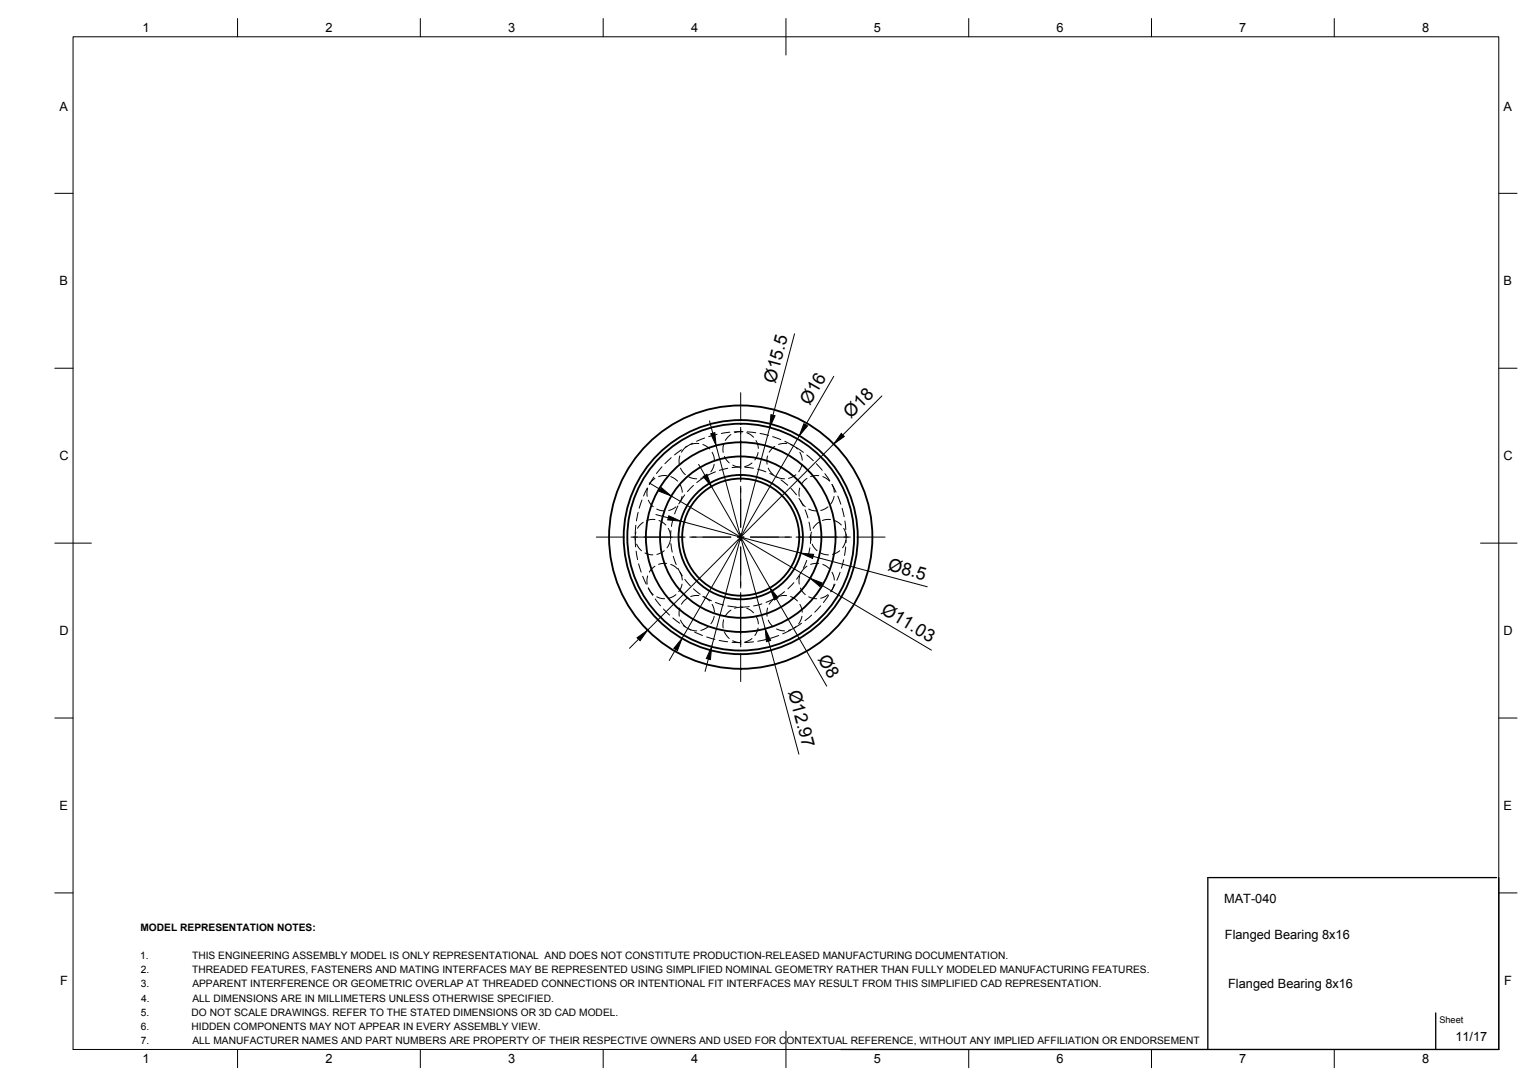
ISO-10303-21;
HEADER;
/* Generated by software containing ST-Developer
 * from STEP Tools, Inc. (www.steptools.com) 
 */

FILE_DESCRIPTION(
/* description */ ('STEP AP214'),
/* implementation_level */ '2;1');

FILE_NAME(
/* name */ 'Flanged Bearing 8x16.step',
/* time_stamp */ '2026-11-14T21:53:28-08:00',
/* author */ (''),
/* organization */ (''),
/* preprocessor_version */ 'ST-DEVELOPER v20.2',
/* originating_system */ 'Autodesk Translation Framework v15.17.0.0',
/* authorisation */ '');

FILE_SCHEMA (('AUTOMOTIVE_DESIGN { 1 0 10303 214 3 1 1 }'));
ENDSEC;

DATA;
#10=MECHANICAL_DESIGN_GEOMETRIC_PRESENTATION_REPRESENTATION('',(#333,#334,#335,#336,#337,#338,#339,#340,#341,#342,#343,#344,#345,#346,#347,#348),#20176);
#215=CONICAL_SURFACE('',#12015,4.25,0.785398163397453);
#216=CONICAL_SURFACE('',#12021,4.,0.785398163397443);
#217=CONICAL_SURFACE('',#12084,8.,0.785398163397446);
#229=TOROIDAL_SURFACE('',#12011,6.,1.21175743903915);
#230=TOROIDAL_SURFACE('',#12075,6.,1.21175743903915);
#252=SPHERICAL_SURFACE('',#12029,1.21175743903915);
#253=SPHERICAL_SURFACE('',#12031,1.21175743903915);
#254=SPHERICAL_SURFACE('',#12033,1.21175743903915);
#255=SPHERICAL_SURFACE('',#12035,1.21175743903915);
#256=SPHERICAL_SURFACE('',#12037,1.21175743903915);
#257=SPHERICAL_SURFACE('',#12039,1.21175743903915);
#258=SPHERICAL_SURFACE('',#12041,1.21175743903915);
#259=SPHERICAL_SURFACE('',#12043,1.21175743903915);
#260=SPHERICAL_SURFACE('',#12045,1.21175743903915);
#261=SPHERICAL_SURFACE('',#12047,1.21175743903915);
#262=SPHERICAL_SURFACE('',#12049,1.21175743903915);
#263=SPHERICAL_SURFACE('',#12051,1.21175743903915);
#301=SHAPE_REPRESENTATION_RELATIONSHIP('SRR','None',#20265,#313);
#313=ADVANCED_BREP_SHAPE_REPRESENTATION('',(#360,#361,#362,#363,#364,#365,
#366,#367,#368,#369,#370,#371,#372,#373,#374,#375),#20171);
#333=STYLED_ITEM('',(#20338),#360);
#334=STYLED_ITEM('',(#20338),#361);
#335=STYLED_ITEM('',(#20338),#362);
#336=STYLED_ITEM('',(#20338),#363);
#337=STYLED_ITEM('',(#20338),#364);
#338=STYLED_ITEM('',(#20338),#365);
#339=STYLED_ITEM('',(#20338),#366);
#340=STYLED_ITEM('',(#20338),#367);
#341=STYLED_ITEM('',(#20338),#368);
#342=STYLED_ITEM('',(#20338),#369);
#343=STYLED_ITEM('',(#20338),#370);
#344=STYLED_ITEM('',(#20338),#371);
#345=STYLED_ITEM('',(#20338),#372);
#346=STYLED_ITEM('',(#20338),#373);
#347=STYLED_ITEM('',(#20338),#374);
#348=STYLED_ITEM('',(#20338),#375);
#360=MANIFOLD_SOLID_BREP('Body1',#10951);
#361=MANIFOLD_SOLID_BREP('Body2',#10952);
#362=MANIFOLD_SOLID_BREP('Body3',#10953);
#363=MANIFOLD_SOLID_BREP('Body4',#10954);
#364=MANIFOLD_SOLID_BREP('Body5',#10955);
#365=MANIFOLD_SOLID_BREP('Body6',#10956);
#366=MANIFOLD_SOLID_BREP('Body7',#10957);
#367=MANIFOLD_SOLID_BREP('Body8',#10958);
#368=MANIFOLD_SOLID_BREP('Body9',#10959);
#369=MANIFOLD_SOLID_BREP('Body10',#10960);
#370=MANIFOLD_SOLID_BREP('Body11',#10961);
#371=MANIFOLD_SOLID_BREP('Body12',#10962);
#372=MANIFOLD_SOLID_BREP('Body13',#10963);
#373=MANIFOLD_SOLID_BREP('Body14',#10964);
#374=MANIFOLD_SOLID_BREP('Body15',#10965);
#375=MANIFOLD_SOLID_BREP('Body16',#10966);
#556=FACE_BOUND('',#2188,.T.);
#557=FACE_BOUND('',#2190,.T.);
#558=FACE_BOUND('',#2206,.T.);
#559=FACE_BOUND('',#2208,.T.);
#560=FACE_BOUND('',#2212,.T.);
#561=FACE_BOUND('',#2214,.T.);
#562=FACE_BOUND('',#2222,.T.);
#563=FACE_BOUND('',#2224,.T.);
#564=FACE_BOUND('',#2226,.T.);
#867=PLANE('',#12027);
#868=PLANE('',#12028);
#869=PLANE('',#12059);
#870=PLANE('',#12060);
#871=PLANE('',#12067);
#872=PLANE('',#12068);
#873=PLANE('',#12086);
#874=PLANE('',#12087);
#875=PLANE('',#12088);
#1413=FACE_OUTER_BOUND('',#2181,.T.);
#1414=FACE_OUTER_BOUND('',#2182,.T.);
#1415=FACE_OUTER_BOUND('',#2183,.T.);
#1416=FACE_OUTER_BOUND('',#2184,.T.);
#1417=FACE_OUTER_BOUND('',#2185,.T.);
#1418=FACE_OUTER_BOUND('',#2186,.T.);
#1419=FACE_OUTER_BOUND('',#2187,.T.);
#1420=FACE_OUTER_BOUND('',#2189,.T.);
#1421=FACE_OUTER_BOUND('',#2191,.T.);
#1422=FACE_OUTER_BOUND('',#2192,.T.);
#1423=FACE_OUTER_BOUND('',#2193,.T.);
#1424=FACE_OUTER_BOUND('',#2194,.T.);
#1425=FACE_OUTER_BOUND('',#2195,.T.);
#1426=FACE_OUTER_BOUND('',#2196,.T.);
#1427=FACE_OUTER_BOUND('',#2197,.T.);
#1428=FACE_OUTER_BOUND('',#2198,.T.);
#1429=FACE_OUTER_BOUND('',#2199,.T.);
#1430=FACE_OUTER_BOUND('',#2200,.T.);
#1431=FACE_OUTER_BOUND('',#2201,.T.);
#1432=FACE_OUTER_BOUND('',#2202,.T.);
#1433=FACE_OUTER_BOUND('',#2203,.T.);
#1434=FACE_OUTER_BOUND('',#2204,.T.);
#1435=FACE_OUTER_BOUND('',#2205,.T.);
#1436=FACE_OUTER_BOUND('',#2207,.T.);
#1437=FACE_OUTER_BOUND('',#2209,.T.);
#1438=FACE_OUTER_BOUND('',#2210,.T.);
#1439=FACE_OUTER_BOUND('',#2211,.T.);
#1440=FACE_OUTER_BOUND('',#2213,.T.);
#1441=FACE_OUTER_BOUND('',#2215,.T.);
#1442=FACE_OUTER_BOUND('',#2216,.T.);
#1443=FACE_OUTER_BOUND('',#2217,.T.);
#1444=FACE_OUTER_BOUND('',#2218,.T.);
#1445=FACE_OUTER_BOUND('',#2219,.T.);
#1446=FACE_OUTER_BOUND('',#2220,.T.);
#1447=FACE_OUTER_BOUND('',#2221,.T.);
#1448=FACE_OUTER_BOUND('',#2223,.T.);
#1449=FACE_OUTER_BOUND('',#2225,.T.);
#2181=EDGE_LOOP('',(#9871,#9872,#9873,#9874));
#2182=EDGE_LOOP('',(#9875,#9876,#9877,#9878));
#2183=EDGE_LOOP('',(#9879,#9880,#9881,#9882,#9883));
#2184=EDGE_LOOP('',(#9884,#9885,#9886,#9887,#9888));
#2185=EDGE_LOOP('',(#9889,#9890,#9891,#9892));
#2186=EDGE_LOOP('',(#9893,#9894,#9895,#9896));
#2187=EDGE_LOOP('',(#9897));
#2188=EDGE_LOOP('',(#9898));
#2189=EDGE_LOOP('',(#9899));
#2190=EDGE_LOOP('',(#9900));
#2191=EDGE_LOOP('',(#9901,#9902));
#2192=EDGE_LOOP('',(#9903,#9904));
#2193=EDGE_LOOP('',(#9905,#9906));
#2194=EDGE_LOOP('',(#9907,#9908));
#2195=EDGE_LOOP('',(#9909,#9910));
#2196=EDGE_LOOP('',(#9911,#9912));
#2197=EDGE_LOOP('',(#9913,#9914));
#2198=EDGE_LOOP('',(#9915,#9916));
#2199=EDGE_LOOP('',(#9917,#9918));
#2200=EDGE_LOOP('',(#9919,#9920));
#2201=EDGE_LOOP('',(#9921,#9922));
#2202=EDGE_LOOP('',(#9923,#9924));
#2203=EDGE_LOOP('',(#9925,#9926,#9927,#9928));
#2204=EDGE_LOOP('',(#9929,#9930,#9931,#9932));
#2205=EDGE_LOOP('',(#9933));
#2206=EDGE_LOOP('',(#9934));
#2207=EDGE_LOOP('',(#9935));
#2208=EDGE_LOOP('',(#9936));
#2209=EDGE_LOOP('',(#9937,#9938,#9939,#9940));
#2210=EDGE_LOOP('',(#9941,#9942,#9943,#9944));
#2211=EDGE_LOOP('',(#9945));
#2212=EDGE_LOOP('',(#9946));
#2213=EDGE_LOOP('',(#9947));
#2214=EDGE_LOOP('',(#9948));
#2215=EDGE_LOOP('',(#9949,#9950,#9951,#9952));
#2216=EDGE_LOOP('',(#9953,#9954,#9955,#9956));
#2217=EDGE_LOOP('',(#9957,#9958,#9959,#9960));
#2218=EDGE_LOOP('',(#9961,#9962,#9963,#9964));
#2219=EDGE_LOOP('',(#9965,#9966,#9967,#9968,#9969));
#2220=EDGE_LOOP('',(#9970,#9971,#9972,#9973,#9974));
#2221=EDGE_LOOP('',(#9975));
#2222=EDGE_LOOP('',(#9976));
#2223=EDGE_LOOP('',(#9977));
#2224=EDGE_LOOP('',(#9978));
#2225=EDGE_LOOP('',(#9979));
#2226=EDGE_LOOP('',(#9980));
#3207=LINE('',#19789,#4195);
#3208=LINE('',#19796,#4196);
#3209=LINE('',#19799,#4197);
#3210=LINE('',#19803,#4198);
#3211=LINE('',#19808,#4199);
#3212=LINE('',#19863,#4200);
#3213=LINE('',#19869,#4201);
#3214=LINE('',#19877,#4202);
#3215=LINE('',#19883,#4203);
#3216=LINE('',#19891,#4204);
#3217=LINE('',#19897,#4205);
#3218=LINE('',#19906,#4206);
#3219=LINE('',#19913,#4207);
#3220=LINE('',#19917,#4208);
#4195=VECTOR('',#14967,4.25);
#4196=VECTOR('',#14976,4.);
#4197=VECTOR('',#14979,4.);
#4198=VECTOR('',#14984,5.51648351648352);
#4199=VECTOR('',#14991,5.51648351648352);
#4200=VECTOR('',#15048,6.48351648351648);
#4201=VECTOR('',#15055,5.51648351648352);
#4202=VECTOR('',#15066,6.48351648351649);
#4203=VECTOR('',#15073,5.51648351648352);
#4204=VECTOR('',#15084,9.);
#4205=VECTOR('',#15091,6.48351648351648);
#4206=VECTOR('',#15104,6.48351648351648);
#4207=VECTOR('',#15111,8.);
#4208=VECTOR('',#15116,8.);
#4651=CIRCLE('',#12012,5.51648351648352);
#4652=CIRCLE('',#12013,1.21175743903915);
#4653=CIRCLE('',#12014,5.51648351648352);
#4654=CIRCLE('',#12016,4.);
#4655=CIRCLE('',#12017,4.25);
#4656=CIRCLE('',#12019,4.);
#4657=CIRCLE('',#12020,4.);
#4658=CIRCLE('',#12022,4.25);
#4659=CIRCLE('',#12024,5.51648351648352);
#4660=CIRCLE('',#12026,5.51648351648352);
#4661=CIRCLE('',#12030,1.21175743903915);
#4662=CIRCLE('',#12032,1.21175743903915);
#4663=CIRCLE('',#12034,1.21175743903915);
#4664=CIRCLE('',#12036,1.21175743903915);
#4665=CIRCLE('',#12038,1.21175743903915);
#4666=CIRCLE('',#12040,1.21175743903915);
#4667=CIRCLE('',#12042,1.21175743903915);
#4668=CIRCLE('',#12044,1.21175743903915);
#4669=CIRCLE('',#12046,1.21175743903915);
#4670=CIRCLE('',#12048,1.21175743903915);
#4671=CIRCLE('',#12050,1.21175743903915);
#4672=CIRCLE('',#12052,1.21175743903915);
#4673=CIRCLE('',#12054,6.48351648351648);
#4674=CIRCLE('',#12055,6.48351648351648);
#4675=CIRCLE('',#12057,5.51648351648352);
#4676=CIRCLE('',#12058,5.51648351648352);
#4677=CIRCLE('',#12062,6.48351648351649);
#4678=CIRCLE('',#12063,6.48351648351649);
#4679=CIRCLE('',#12065,5.51648351648352);
#4680=CIRCLE('',#12066,5.51648351648352);
#4681=CIRCLE('',#12070,9.);
#4682=CIRCLE('',#12071,9.);
#4683=CIRCLE('',#12073,6.48351648351648);
#4684=CIRCLE('',#12074,6.48351648351648);
#4685=CIRCLE('',#12076,6.48351648351648);
#4686=CIRCLE('',#12077,1.21175743903915);
#4687=CIRCLE('',#12079,6.48351648351649);
#4688=CIRCLE('',#12081,8.);
#4689=CIRCLE('',#12082,8.);
#4690=CIRCLE('',#12083,8.);
#4691=CIRCLE('',#12085,7.75);
#5592=VERTEX_POINT('',#19780);
#5593=VERTEX_POINT('',#19782);
#5594=VERTEX_POINT('',#19786);
#5595=VERTEX_POINT('',#19788);
#5596=VERTEX_POINT('',#19792);
#5597=VERTEX_POINT('',#19793);
#5598=VERTEX_POINT('',#19798);
#5599=VERTEX_POINT('',#19802);
#5600=VERTEX_POINT('',#19806);
#5601=VERTEX_POINT('',#19812);
#5602=VERTEX_POINT('',#19813);
#5603=VERTEX_POINT('',#19816);
#5604=VERTEX_POINT('',#19817);
#5605=VERTEX_POINT('',#19820);
#5606=VERTEX_POINT('',#19821);
#5607=VERTEX_POINT('',#19824);
#5608=VERTEX_POINT('',#19825);
#5609=VERTEX_POINT('',#19828);
#5610=VERTEX_POINT('',#19829);
#5611=VERTEX_POINT('',#19832);
#5612=VERTEX_POINT('',#19833);
#5613=VERTEX_POINT('',#19836);
#5614=VERTEX_POINT('',#19837);
#5615=VERTEX_POINT('',#19840);
#5616=VERTEX_POINT('',#19841);
#5617=VERTEX_POINT('',#19844);
#5618=VERTEX_POINT('',#19845);
#5619=VERTEX_POINT('',#19848);
#5620=VERTEX_POINT('',#19849);
#5621=VERTEX_POINT('',#19852);
#5622=VERTEX_POINT('',#19853);
#5623=VERTEX_POINT('',#19856);
#5624=VERTEX_POINT('',#19857);
#5625=VERTEX_POINT('',#19860);
#5626=VERTEX_POINT('',#19862);
#5627=VERTEX_POINT('',#19866);
#5628=VERTEX_POINT('',#19868);
#5629=VERTEX_POINT('',#19874);
#5630=VERTEX_POINT('',#19876);
#5631=VERTEX_POINT('',#19880);
#5632=VERTEX_POINT('',#19882);
#5633=VERTEX_POINT('',#19888);
#5634=VERTEX_POINT('',#19890);
#5635=VERTEX_POINT('',#19894);
#5636=VERTEX_POINT('',#19896);
#5637=VERTEX_POINT('',#19900);
#5638=VERTEX_POINT('',#19904);
#5639=VERTEX_POINT('',#19908);
#5640=VERTEX_POINT('',#19909);
#5641=VERTEX_POINT('',#19912);
#5642=VERTEX_POINT('',#19916);
#7046=EDGE_CURVE('',#5592,#5592,#4651,.T.);
#7047=EDGE_CURVE('',#5592,#5593,#4652,.T.);
#7048=EDGE_CURVE('',#5593,#5593,#4653,.T.);
#7049=EDGE_CURVE('',#5594,#5594,#4654,.T.);
#7050=EDGE_CURVE('',#5594,#5595,#3207,.T.);
#7051=EDGE_CURVE('',#5595,#5595,#4655,.T.);
#7052=EDGE_CURVE('',#5596,#5597,#4656,.T.);
#7053=EDGE_CURVE('',#5597,#5596,#4657,.T.);
#7054=EDGE_CURVE('',#5597,#5594,#3208,.T.);
#7055=EDGE_CURVE('',#5596,#5598,#3209,.T.);
#7056=EDGE_CURVE('',#5598,#5598,#4658,.T.);
#7057=EDGE_CURVE('',#5593,#5599,#3210,.T.);
#7058=EDGE_CURVE('',#5599,#5599,#4659,.T.);
#7059=EDGE_CURVE('',#5600,#5600,#4660,.T.);
#7060=EDGE_CURVE('',#5600,#5592,#3211,.T.);
#7061=EDGE_CURVE('',#5601,#5602,#4661,.T.);
#7062=EDGE_CURVE('',#5603,#5604,#4662,.T.);
#7063=EDGE_CURVE('',#5605,#5606,#4663,.T.);
#7064=EDGE_CURVE('',#5607,#5608,#4664,.T.);
#7065=EDGE_CURVE('',#5609,#5610,#4665,.T.);
#7066=EDGE_CURVE('',#5611,#5612,#4666,.T.);
#7067=EDGE_CURVE('',#5613,#5614,#4667,.T.);
#7068=EDGE_CURVE('',#5615,#5616,#4668,.T.);
#7069=EDGE_CURVE('',#5617,#5618,#4669,.T.);
#7070=EDGE_CURVE('',#5619,#5620,#4670,.T.);
#7071=EDGE_CURVE('',#5621,#5622,#4671,.T.);
#7072=EDGE_CURVE('',#5623,#5624,#4672,.T.);
#7073=EDGE_CURVE('',#5625,#5625,#4673,.T.);
#7074=EDGE_CURVE('',#5625,#5626,#3212,.T.);
#7075=EDGE_CURVE('',#5626,#5626,#4674,.T.);
#7076=EDGE_CURVE('',#5627,#5627,#4675,.T.);
#7077=EDGE_CURVE('',#5627,#5628,#3213,.T.);
#7078=EDGE_CURVE('',#5628,#5628,#4676,.T.);
#7079=EDGE_CURVE('',#5629,#5629,#4677,.T.);
#7080=EDGE_CURVE('',#5629,#5630,#3214,.T.);
#7081=EDGE_CURVE('',#5630,#5630,#4678,.T.);
#7082=EDGE_CURVE('',#5631,#5631,#4679,.T.);
#7083=EDGE_CURVE('',#5631,#5632,#3215,.T.);
#7084=EDGE_CURVE('',#5632,#5632,#4680,.T.);
#7085=EDGE_CURVE('',#5633,#5633,#4681,.T.);
#7086=EDGE_CURVE('',#5633,#5634,#3216,.T.);
#7087=EDGE_CURVE('',#5634,#5634,#4682,.T.);
#7088=EDGE_CURVE('',#5635,#5635,#4683,.T.);
#7089=EDGE_CURVE('',#5635,#5636,#3217,.T.);
#7090=EDGE_CURVE('',#5636,#5636,#4684,.T.);
#7091=EDGE_CURVE('',#5637,#5637,#4685,.T.);
#7092=EDGE_CURVE('',#5637,#5635,#4686,.T.);
#7093=EDGE_CURVE('',#5638,#5638,#4687,.T.);
#7094=EDGE_CURVE('',#5638,#5637,#3218,.T.);
#7095=EDGE_CURVE('',#5639,#5640,#4688,.T.);
#7096=EDGE_CURVE('',#5640,#5639,#4689,.T.);
#7097=EDGE_CURVE('',#5640,#5641,#3219,.T.);
#7098=EDGE_CURVE('',#5641,#5641,#4690,.T.);
#7099=EDGE_CURVE('',#5639,#5642,#3220,.T.);
#7100=EDGE_CURVE('',#5642,#5642,#4691,.T.);
#9871=ORIENTED_EDGE('',*,*,#7046,.F.);
#9872=ORIENTED_EDGE('',*,*,#7047,.T.);
#9873=ORIENTED_EDGE('',*,*,#7048,.T.);
#9874=ORIENTED_EDGE('',*,*,#7047,.F.);
#9875=ORIENTED_EDGE('',*,*,#7049,.F.);
#9876=ORIENTED_EDGE('',*,*,#7050,.T.);
#9877=ORIENTED_EDGE('',*,*,#7051,.T.);
#9878=ORIENTED_EDGE('',*,*,#7050,.F.);
#9879=ORIENTED_EDGE('',*,*,#7052,.F.);
#9880=ORIENTED_EDGE('',*,*,#7053,.F.);
#9881=ORIENTED_EDGE('',*,*,#7054,.T.);
#9882=ORIENTED_EDGE('',*,*,#7049,.T.);
#9883=ORIENTED_EDGE('',*,*,#7054,.F.);
#9884=ORIENTED_EDGE('',*,*,#7052,.T.);
#9885=ORIENTED_EDGE('',*,*,#7053,.T.);
#9886=ORIENTED_EDGE('',*,*,#7055,.T.);
#9887=ORIENTED_EDGE('',*,*,#7056,.F.);
#9888=ORIENTED_EDGE('',*,*,#7055,.F.);
#9889=ORIENTED_EDGE('',*,*,#7048,.F.);
#9890=ORIENTED_EDGE('',*,*,#7057,.T.);
#9891=ORIENTED_EDGE('',*,*,#7058,.T.);
#9892=ORIENTED_EDGE('',*,*,#7057,.F.);
#9893=ORIENTED_EDGE('',*,*,#7059,.F.);
#9894=ORIENTED_EDGE('',*,*,#7060,.T.);
#9895=ORIENTED_EDGE('',*,*,#7046,.T.);
#9896=ORIENTED_EDGE('',*,*,#7060,.F.);
#9897=ORIENTED_EDGE('',*,*,#7059,.T.);
#9898=ORIENTED_EDGE('',*,*,#7051,.F.);
#9899=ORIENTED_EDGE('',*,*,#7058,.F.);
#9900=ORIENTED_EDGE('',*,*,#7056,.T.);
#9901=ORIENTED_EDGE('',*,*,#7061,.T.);
#9902=ORIENTED_EDGE('',*,*,#7061,.F.);
#9903=ORIENTED_EDGE('',*,*,#7062,.T.);
#9904=ORIENTED_EDGE('',*,*,#7062,.F.);
#9905=ORIENTED_EDGE('',*,*,#7063,.T.);
#9906=ORIENTED_EDGE('',*,*,#7063,.F.);
#9907=ORIENTED_EDGE('',*,*,#7064,.T.);
#9908=ORIENTED_EDGE('',*,*,#7064,.F.);
#9909=ORIENTED_EDGE('',*,*,#7065,.T.);
#9910=ORIENTED_EDGE('',*,*,#7065,.F.);
#9911=ORIENTED_EDGE('',*,*,#7066,.T.);
#9912=ORIENTED_EDGE('',*,*,#7066,.F.);
#9913=ORIENTED_EDGE('',*,*,#7067,.T.);
#9914=ORIENTED_EDGE('',*,*,#7067,.F.);
#9915=ORIENTED_EDGE('',*,*,#7068,.T.);
#9916=ORIENTED_EDGE('',*,*,#7068,.F.);
#9917=ORIENTED_EDGE('',*,*,#7069,.T.);
#9918=ORIENTED_EDGE('',*,*,#7069,.F.);
#9919=ORIENTED_EDGE('',*,*,#7070,.T.);
#9920=ORIENTED_EDGE('',*,*,#7070,.F.);
#9921=ORIENTED_EDGE('',*,*,#7071,.T.);
#9922=ORIENTED_EDGE('',*,*,#7071,.F.);
#9923=ORIENTED_EDGE('',*,*,#7072,.T.);
#9924=ORIENTED_EDGE('',*,*,#7072,.F.);
#9925=ORIENTED_EDGE('',*,*,#7073,.F.);
#9926=ORIENTED_EDGE('',*,*,#7074,.T.);
#9927=ORIENTED_EDGE('',*,*,#7075,.T.);
#9928=ORIENTED_EDGE('',*,*,#7074,.F.);
#9929=ORIENTED_EDGE('',*,*,#7076,.F.);
#9930=ORIENTED_EDGE('',*,*,#7077,.T.);
#9931=ORIENTED_EDGE('',*,*,#7078,.T.);
#9932=ORIENTED_EDGE('',*,*,#7077,.F.);
#9933=ORIENTED_EDGE('',*,*,#7073,.T.);
#9934=ORIENTED_EDGE('',*,*,#7078,.F.);
#9935=ORIENTED_EDGE('',*,*,#7075,.F.);
#9936=ORIENTED_EDGE('',*,*,#7076,.T.);
#9937=ORIENTED_EDGE('',*,*,#7079,.F.);
#9938=ORIENTED_EDGE('',*,*,#7080,.T.);
#9939=ORIENTED_EDGE('',*,*,#7081,.T.);
#9940=ORIENTED_EDGE('',*,*,#7080,.F.);
#9941=ORIENTED_EDGE('',*,*,#7082,.F.);
#9942=ORIENTED_EDGE('',*,*,#7083,.T.);
#9943=ORIENTED_EDGE('',*,*,#7084,.T.);
#9944=ORIENTED_EDGE('',*,*,#7083,.F.);
#9945=ORIENTED_EDGE('',*,*,#7081,.F.);
#9946=ORIENTED_EDGE('',*,*,#7082,.T.);
#9947=ORIENTED_EDGE('',*,*,#7079,.T.);
#9948=ORIENTED_EDGE('',*,*,#7084,.F.);
#9949=ORIENTED_EDGE('',*,*,#7085,.F.);
#9950=ORIENTED_EDGE('',*,*,#7086,.T.);
#9951=ORIENTED_EDGE('',*,*,#7087,.T.);
#9952=ORIENTED_EDGE('',*,*,#7086,.F.);
#9953=ORIENTED_EDGE('',*,*,#7088,.F.);
#9954=ORIENTED_EDGE('',*,*,#7089,.T.);
#9955=ORIENTED_EDGE('',*,*,#7090,.T.);
#9956=ORIENTED_EDGE('',*,*,#7089,.F.);
#9957=ORIENTED_EDGE('',*,*,#7091,.F.);
#9958=ORIENTED_EDGE('',*,*,#7092,.T.);
#9959=ORIENTED_EDGE('',*,*,#7088,.T.);
#9960=ORIENTED_EDGE('',*,*,#7092,.F.);
#9961=ORIENTED_EDGE('',*,*,#7093,.F.);
#9962=ORIENTED_EDGE('',*,*,#7094,.T.);
#9963=ORIENTED_EDGE('',*,*,#7091,.T.);
#9964=ORIENTED_EDGE('',*,*,#7094,.F.);
#9965=ORIENTED_EDGE('',*,*,#7095,.F.);
#9966=ORIENTED_EDGE('',*,*,#7096,.F.);
#9967=ORIENTED_EDGE('',*,*,#7097,.T.);
#9968=ORIENTED_EDGE('',*,*,#7098,.T.);
#9969=ORIENTED_EDGE('',*,*,#7097,.F.);
#9970=ORIENTED_EDGE('',*,*,#7095,.T.);
#9971=ORIENTED_EDGE('',*,*,#7096,.T.);
#9972=ORIENTED_EDGE('',*,*,#7099,.T.);
#9973=ORIENTED_EDGE('',*,*,#7100,.F.);
#9974=ORIENTED_EDGE('',*,*,#7099,.F.);
#9975=ORIENTED_EDGE('',*,*,#7085,.T.);
#9976=ORIENTED_EDGE('',*,*,#7093,.T.);
#9977=ORIENTED_EDGE('',*,*,#7100,.T.);
#9978=ORIENTED_EDGE('',*,*,#7090,.F.);
#9979=ORIENTED_EDGE('',*,*,#7087,.F.);
#9980=ORIENTED_EDGE('',*,*,#7098,.F.);
#10329=CYLINDRICAL_SURFACE('',#12018,4.);
#10330=CYLINDRICAL_SURFACE('',#12023,5.51648351648352);
#10331=CYLINDRICAL_SURFACE('',#12025,5.51648351648352);
#10332=CYLINDRICAL_SURFACE('',#12053,6.48351648351648);
#10333=CYLINDRICAL_SURFACE('',#12056,5.51648351648352);
#10334=CYLINDRICAL_SURFACE('',#12061,6.48351648351649);
#10335=CYLINDRICAL_SURFACE('',#12064,5.51648351648352);
#10336=CYLINDRICAL_SURFACE('',#12069,9.);
#10337=CYLINDRICAL_SURFACE('',#12072,6.48351648351648);
#10338=CYLINDRICAL_SURFACE('',#12078,6.48351648351648);
#10339=CYLINDRICAL_SURFACE('',#12080,8.);
#10865=ADVANCED_FACE('',(#1413),#229,.F.);
#10866=ADVANCED_FACE('',(#1414),#215,.F.);
#10867=ADVANCED_FACE('',(#1415),#10329,.F.);
#10868=ADVANCED_FACE('',(#1416),#216,.F.);
#10869=ADVANCED_FACE('',(#1417),#10330,.T.);
#10870=ADVANCED_FACE('',(#1418),#10331,.T.);
#10871=ADVANCED_FACE('',(#1419,#556),#867,.F.);
#10872=ADVANCED_FACE('',(#1420,#557),#868,.F.);
#10873=ADVANCED_FACE('',(#1421),#252,.T.);
#10874=ADVANCED_FACE('',(#1422),#253,.T.);
#10875=ADVANCED_FACE('',(#1423),#254,.T.);
#10876=ADVANCED_FACE('',(#1424),#255,.T.);
#10877=ADVANCED_FACE('',(#1425),#256,.T.);
#10878=ADVANCED_FACE('',(#1426),#257,.T.);
#10879=ADVANCED_FACE('',(#1427),#258,.T.);
#10880=ADVANCED_FACE('',(#1428),#259,.T.);
#10881=ADVANCED_FACE('',(#1429),#260,.T.);
#10882=ADVANCED_FACE('',(#1430),#261,.T.);
#10883=ADVANCED_FACE('',(#1431),#262,.T.);
#10884=ADVANCED_FACE('',(#1432),#263,.T.);
#10885=ADVANCED_FACE('',(#1433),#10332,.T.);
#10886=ADVANCED_FACE('',(#1434),#10333,.F.);
#10887=ADVANCED_FACE('',(#1435,#558),#869,.F.);
#10888=ADVANCED_FACE('',(#1436,#559),#870,.F.);
#10889=ADVANCED_FACE('',(#1437),#10334,.T.);
#10890=ADVANCED_FACE('',(#1438),#10335,.F.);
#10891=ADVANCED_FACE('',(#1439,#560),#871,.F.);
#10892=ADVANCED_FACE('',(#1440,#561),#872,.F.);
#10893=ADVANCED_FACE('',(#1441),#10336,.T.);
#10894=ADVANCED_FACE('',(#1442),#10337,.F.);
#10895=ADVANCED_FACE('',(#1443),#230,.F.);
#10896=ADVANCED_FACE('',(#1444),#10338,.F.);
#10897=ADVANCED_FACE('',(#1445),#10339,.T.);
#10898=ADVANCED_FACE('',(#1446),#217,.T.);
#10899=ADVANCED_FACE('',(#1447,#562),#873,.F.);
#10900=ADVANCED_FACE('',(#1448,#563),#874,.F.);
#10901=ADVANCED_FACE('',(#1449,#564),#875,.T.);
#10951=CLOSED_SHELL('',(#10865,#10866,#10867,#10868,#10869,#10870,#10871,
#10872));
#10952=CLOSED_SHELL('',(#10873));
#10953=CLOSED_SHELL('',(#10874));
#10954=CLOSED_SHELL('',(#10875));
#10955=CLOSED_SHELL('',(#10876));
#10956=CLOSED_SHELL('',(#10877));
#10957=CLOSED_SHELL('',(#10878));
#10958=CLOSED_SHELL('',(#10879));
#10959=CLOSED_SHELL('',(#10880));
#10960=CLOSED_SHELL('',(#10881));
#10961=CLOSED_SHELL('',(#10882));
#10962=CLOSED_SHELL('',(#10883));
#10963=CLOSED_SHELL('',(#10884));
#10964=CLOSED_SHELL('',(#10885,#10886,#10887,#10888));
#10965=CLOSED_SHELL('',(#10889,#10890,#10891,#10892));
#10966=CLOSED_SHELL('',(#10893,#10894,#10895,#10896,#10897,#10898,#10899,
#10900,#10901));
#12010=AXIS2_PLACEMENT_3D('',#19778,#14953,#14954);
#12011=AXIS2_PLACEMENT_3D('',#19779,#14955,#14956);
#12012=AXIS2_PLACEMENT_3D('',#19781,#14957,#14958);
#12013=AXIS2_PLACEMENT_3D('',#19783,#14959,#14960);
#12014=AXIS2_PLACEMENT_3D('',#19784,#14961,#14962);
#12015=AXIS2_PLACEMENT_3D('',#19785,#14963,#14964);
#12016=AXIS2_PLACEMENT_3D('',#19787,#14965,#14966);
#12017=AXIS2_PLACEMENT_3D('',#19790,#14968,#14969);
#12018=AXIS2_PLACEMENT_3D('',#19791,#14970,#14971);
#12019=AXIS2_PLACEMENT_3D('',#19794,#14972,#14973);
#12020=AXIS2_PLACEMENT_3D('',#19795,#14974,#14975);
#12021=AXIS2_PLACEMENT_3D('',#19797,#14977,#14978);
#12022=AXIS2_PLACEMENT_3D('',#19800,#14980,#14981);
#12023=AXIS2_PLACEMENT_3D('',#19801,#14982,#14983);
#12024=AXIS2_PLACEMENT_3D('',#19804,#14985,#14986);
#12025=AXIS2_PLACEMENT_3D('',#19805,#14987,#14988);
#12026=AXIS2_PLACEMENT_3D('',#19807,#14989,#14990);
#12027=AXIS2_PLACEMENT_3D('',#19809,#14992,#14993);
#12028=AXIS2_PLACEMENT_3D('',#19810,#14994,#14995);
#12029=AXIS2_PLACEMENT_3D('',#19811,#14996,#14997);
#12030=AXIS2_PLACEMENT_3D('',#19814,#14998,#14999);
#12031=AXIS2_PLACEMENT_3D('',#19815,#15000,#15001);
#12032=AXIS2_PLACEMENT_3D('',#19818,#15002,#15003);
#12033=AXIS2_PLACEMENT_3D('',#19819,#15004,#15005);
#12034=AXIS2_PLACEMENT_3D('',#19822,#15006,#15007);
#12035=AXIS2_PLACEMENT_3D('',#19823,#15008,#15009);
#12036=AXIS2_PLACEMENT_3D('',#19826,#15010,#15011);
#12037=AXIS2_PLACEMENT_3D('',#19827,#15012,#15013);
#12038=AXIS2_PLACEMENT_3D('',#19830,#15014,#15015);
#12039=AXIS2_PLACEMENT_3D('',#19831,#15016,#15017);
#12040=AXIS2_PLACEMENT_3D('',#19834,#15018,#15019);
#12041=AXIS2_PLACEMENT_3D('',#19835,#15020,#15021);
#12042=AXIS2_PLACEMENT_3D('',#19838,#15022,#15023);
#12043=AXIS2_PLACEMENT_3D('',#19839,#15024,#15025);
#12044=AXIS2_PLACEMENT_3D('',#19842,#15026,#15027);
#12045=AXIS2_PLACEMENT_3D('',#19843,#15028,#15029);
#12046=AXIS2_PLACEMENT_3D('',#19846,#15030,#15031);
#12047=AXIS2_PLACEMENT_3D('',#19847,#15032,#15033);
#12048=AXIS2_PLACEMENT_3D('',#19850,#15034,#15035);
#12049=AXIS2_PLACEMENT_3D('',#19851,#15036,#15037);
#12050=AXIS2_PLACEMENT_3D('',#19854,#15038,#15039);
#12051=AXIS2_PLACEMENT_3D('',#19855,#15040,#15041);
#12052=AXIS2_PLACEMENT_3D('',#19858,#15042,#15043);
#12053=AXIS2_PLACEMENT_3D('',#19859,#15044,#15045);
#12054=AXIS2_PLACEMENT_3D('',#19861,#15046,#15047);
#12055=AXIS2_PLACEMENT_3D('',#19864,#15049,#15050);
#12056=AXIS2_PLACEMENT_3D('',#19865,#15051,#15052);
#12057=AXIS2_PLACEMENT_3D('',#19867,#15053,#15054);
#12058=AXIS2_PLACEMENT_3D('',#19870,#15056,#15057);
#12059=AXIS2_PLACEMENT_3D('',#19871,#15058,#15059);
#12060=AXIS2_PLACEMENT_3D('',#19872,#15060,#15061);
#12061=AXIS2_PLACEMENT_3D('',#19873,#15062,#15063);
#12062=AXIS2_PLACEMENT_3D('',#19875,#15064,#15065);
#12063=AXIS2_PLACEMENT_3D('',#19878,#15067,#15068);
#12064=AXIS2_PLACEMENT_3D('',#19879,#15069,#15070);
#12065=AXIS2_PLACEMENT_3D('',#19881,#15071,#15072);
#12066=AXIS2_PLACEMENT_3D('',#19884,#15074,#15075);
#12067=AXIS2_PLACEMENT_3D('',#19885,#15076,#15077);
#12068=AXIS2_PLACEMENT_3D('',#19886,#15078,#15079);
#12069=AXIS2_PLACEMENT_3D('',#19887,#15080,#15081);
#12070=AXIS2_PLACEMENT_3D('',#19889,#15082,#15083);
#12071=AXIS2_PLACEMENT_3D('',#19892,#15085,#15086);
#12072=AXIS2_PLACEMENT_3D('',#19893,#15087,#15088);
#12073=AXIS2_PLACEMENT_3D('',#19895,#15089,#15090);
#12074=AXIS2_PLACEMENT_3D('',#19898,#15092,#15093);
#12075=AXIS2_PLACEMENT_3D('',#19899,#15094,#15095);
#12076=AXIS2_PLACEMENT_3D('',#19901,#15096,#15097);
#12077=AXIS2_PLACEMENT_3D('',#19902,#15098,#15099);
#12078=AXIS2_PLACEMENT_3D('',#19903,#15100,#15101);
#12079=AXIS2_PLACEMENT_3D('',#19905,#15102,#15103);
#12080=AXIS2_PLACEMENT_3D('',#19907,#15105,#15106);
#12081=AXIS2_PLACEMENT_3D('',#19910,#15107,#15108);
#12082=AXIS2_PLACEMENT_3D('',#19911,#15109,#15110);
#12083=AXIS2_PLACEMENT_3D('',#19914,#15112,#15113);
#12084=AXIS2_PLACEMENT_3D('',#19915,#15114,#15115);
#12085=AXIS2_PLACEMENT_3D('',#19918,#15117,#15118);
#12086=AXIS2_PLACEMENT_3D('',#19919,#15119,#15120);
#12087=AXIS2_PLACEMENT_3D('',#19920,#15121,#15122);
#12088=AXIS2_PLACEMENT_3D('',#19921,#15123,#15124);
#14953=DIRECTION('axis',(0.,0.,1.));
#14954=DIRECTION('refdir',(1.,0.,0.));
#14955=DIRECTION('center_axis',(0.,0.,1.));
#14956=DIRECTION('ref_axis',(1.,0.,0.));
#14957=DIRECTION('center_axis',(0.,0.,1.));
#14958=DIRECTION('ref_axis',(1.,0.,0.));
#14959=DIRECTION('center_axis',(-1.22464679914735E-16,1.,0.));
#14960=DIRECTION('ref_axis',(-1.,-1.22464679914735E-16,0.));
#14961=DIRECTION('center_axis',(0.,0.,1.));
#14962=DIRECTION('ref_axis',(1.,0.,0.));
#14963=DIRECTION('center_axis',(0.,0.,1.));
#14964=DIRECTION('ref_axis',(1.,0.,0.));
#14965=DIRECTION('center_axis',(0.,0.,1.));
#14966=DIRECTION('ref_axis',(1.,0.,0.));
#14967=DIRECTION('',(-0.707106781186551,-8.65956056235498E-17,0.707106781186544));
#14968=DIRECTION('center_axis',(0.,0.,1.));
#14969=DIRECTION('ref_axis',(1.,0.,0.));
#14970=DIRECTION('center_axis',(0.,0.,1.));
#14971=DIRECTION('ref_axis',(1.,0.,0.));
#14972=DIRECTION('center_axis',(0.,0.,1.));
#14973=DIRECTION('ref_axis',(1.,0.,0.));
#14974=DIRECTION('center_axis',(0.,0.,1.));
#14975=DIRECTION('ref_axis',(1.,0.,0.));
#14976=DIRECTION('',(0.,0.,1.));
#14977=DIRECTION('center_axis',(0.,0.,-1.));
#14978=DIRECTION('ref_axis',(-1.,0.,0.));
#14979=DIRECTION('',(0.707106781186544,-8.65956056235489E-17,-0.707106781186551));
#14980=DIRECTION('center_axis',(0.,0.,1.));
#14981=DIRECTION('ref_axis',(1.,0.,0.));
#14982=DIRECTION('center_axis',(0.,0.,1.));
#14983=DIRECTION('ref_axis',(1.,0.,0.));
#14984=DIRECTION('',(0.,0.,-1.));
#14985=DIRECTION('center_axis',(0.,0.,1.));
#14986=DIRECTION('ref_axis',(1.,0.,0.));
#14987=DIRECTION('center_axis',(0.,0.,1.));
#14988=DIRECTION('ref_axis',(1.,0.,0.));
#14989=DIRECTION('center_axis',(0.,0.,1.));
#14990=DIRECTION('ref_axis',(1.,0.,0.));
#14991=DIRECTION('',(0.,0.,-1.));
#14992=DIRECTION('center_axis',(0.,0.,-1.));
#14993=DIRECTION('ref_axis',(-1.,0.,0.));
#14994=DIRECTION('center_axis',(0.,0.,1.));
#14995=DIRECTION('ref_axis',(1.,0.,0.));
#14996=DIRECTION('center_axis',(-1.,0.,0.));
#14997=DIRECTION('ref_axis',(0.,1.,0.));
#14998=DIRECTION('center_axis',(0.,1.22464679914735E-16,1.));
#14999=DIRECTION('ref_axis',(0.,-1.,1.22464679914735E-16));
#15000=DIRECTION('center_axis',(-0.866025403784438,0.500000000000001,0.));
#15001=DIRECTION('ref_axis',(0.500000000000001,0.866025403784438,0.));
#15002=DIRECTION('center_axis',(6.12323399573678E-17,1.06057523872491E-16,
1.));
#15003=DIRECTION('ref_axis',(-0.500000000000001,-0.866025403784438,1.22464679914735E-16));
#15004=DIRECTION('center_axis',(-0.499999999999998,0.86602540378444,0.));
#15005=DIRECTION('ref_axis',(0.86602540378444,0.499999999999998,0.));
#15006=DIRECTION('center_axis',(1.06057523872491E-16,6.12323399573674E-17,
1.));
#15007=DIRECTION('ref_axis',(-0.86602540378444,-0.499999999999998,1.22464679914735E-16));
#15008=DIRECTION('center_axis',(3.66483584538337E-15,1.,0.));
#15009=DIRECTION('ref_axis',(1.,-3.49148336110938E-15,0.));
#15010=DIRECTION('center_axis',(1.22464679914735E-16,-4.27583392245885E-31,
1.));
#15011=DIRECTION('ref_axis',(-1.,3.49148336110938E-15,1.22464679914735E-16));
#15012=DIRECTION('center_axis',(0.500000000000004,0.866025403784436,0.));
#15013=DIRECTION('ref_axis',(0.866025403784436,-0.500000000000004,0.));
#15014=DIRECTION('center_axis',(1.0605752387249E-16,-6.12323399573681E-17,
1.));
#15015=DIRECTION('ref_axis',(-0.866025403784436,0.500000000000004,1.22464679914735E-16));
#15016=DIRECTION('center_axis',(0.866025403784441,0.499999999999995,0.));
#15017=DIRECTION('ref_axis',(0.499999999999995,-0.866025403784441,0.));
#15018=DIRECTION('center_axis',(6.1232339957367E-17,-1.06057523872491E-16,
1.));
#15019=DIRECTION('ref_axis',(-0.499999999999995,0.866025403784441,1.22464679914735E-16));
#15020=DIRECTION('center_axis',(1.,-7.32967169076675E-15,0.));
#15021=DIRECTION('ref_axis',(-6.98296672221876E-15,-1.,0.));
#15022=DIRECTION('center_axis',(-8.55166784491769E-31,-1.22464679914735E-16,
1.));
#15023=DIRECTION('ref_axis',(6.98296672221877E-15,1.,1.22464679914735E-16));
#15024=DIRECTION('center_axis',(0.866025403784434,-0.500000000000008,0.));
#15025=DIRECTION('ref_axis',(-0.500000000000008,-0.866025403784434,0.));
#15026=DIRECTION('center_axis',(-6.12323399573685E-17,-1.0605752387249E-16,
1.));
#15027=DIRECTION('ref_axis',(0.500000000000007,0.866025403784434,1.22464679914735E-16));
#15028=DIRECTION('center_axis',(0.499999999999992,-0.866025403784443,0.));
#15029=DIRECTION('ref_axis',(-0.866025403784443,-0.499999999999992,0.));
#15030=DIRECTION('center_axis',(-1.06057523872491E-16,-6.12323399573666E-17,
1.));
#15031=DIRECTION('ref_axis',(0.866025403784443,0.499999999999992,1.22464679914735E-16));
#15032=DIRECTION('center_axis',(-1.02615403670734E-14,-1.,0.));
#15033=DIRECTION('ref_axis',(-1.,1.04744500833281E-14,0.));
#15034=DIRECTION('center_axis',(-1.22464679914735E-16,1.28275017673765E-30,
1.));
#15035=DIRECTION('ref_axis',(1.,-1.04744500833281E-14,1.22464679914735E-16));
#15036=DIRECTION('center_axis',(-0.50000000000001,-0.866025403784433,0.));
#15037=DIRECTION('ref_axis',(-0.866025403784433,0.50000000000001,0.));
#15038=DIRECTION('center_axis',(-1.0605752387249E-16,6.12323399573689E-17,
1.));
#15039=DIRECTION('ref_axis',(0.866025403784433,-0.50000000000001,1.22464679914735E-16));
#15040=DIRECTION('center_axis',(-0.866025403784445,-0.499999999999989,0.));
#15041=DIRECTION('ref_axis',(-0.499999999999989,0.866025403784445,0.));
#15042=DIRECTION('center_axis',(-6.12323399573663E-17,1.06057523872491E-16,
1.));
#15043=DIRECTION('ref_axis',(0.499999999999989,-0.866025403784445,1.22464679914735E-16));
#15044=DIRECTION('center_axis',(0.,0.,1.));
#15045=DIRECTION('ref_axis',(1.,0.,0.));
#15046=DIRECTION('center_axis',(0.,0.,1.));
#15047=DIRECTION('ref_axis',(1.,0.,0.));
#15048=DIRECTION('',(0.,0.,-1.));
#15049=DIRECTION('center_axis',(0.,0.,1.));
#15050=DIRECTION('ref_axis',(1.,0.,0.));
#15051=DIRECTION('center_axis',(0.,0.,1.));
#15052=DIRECTION('ref_axis',(1.,0.,0.));
#15053=DIRECTION('center_axis',(0.,0.,1.));
#15054=DIRECTION('ref_axis',(1.,0.,0.));
#15055=DIRECTION('',(0.,0.,1.));
#15056=DIRECTION('center_axis',(0.,0.,1.));
#15057=DIRECTION('ref_axis',(1.,0.,0.));
#15058=DIRECTION('center_axis',(0.,0.,-1.));
#15059=DIRECTION('ref_axis',(-1.,0.,0.));
#15060=DIRECTION('center_axis',(0.,0.,1.));
#15061=DIRECTION('ref_axis',(1.,0.,0.));
#15062=DIRECTION('center_axis',(0.,0.,1.));
#15063=DIRECTION('ref_axis',(1.,0.,0.));
#15064=DIRECTION('center_axis',(0.,0.,1.));
#15065=DIRECTION('ref_axis',(1.,0.,0.));
#15066=DIRECTION('',(0.,0.,-1.));
#15067=DIRECTION('center_axis',(0.,0.,1.));
#15068=DIRECTION('ref_axis',(1.,0.,0.));
#15069=DIRECTION('center_axis',(0.,0.,1.));
#15070=DIRECTION('ref_axis',(1.,0.,0.));
#15071=DIRECTION('center_axis',(0.,0.,1.));
#15072=DIRECTION('ref_axis',(1.,0.,0.));
#15073=DIRECTION('',(0.,0.,1.));
#15074=DIRECTION('center_axis',(0.,0.,1.));
#15075=DIRECTION('ref_axis',(1.,0.,0.));
#15076=DIRECTION('center_axis',(0.,0.,1.));
#15077=DIRECTION('ref_axis',(1.,0.,0.));
#15078=DIRECTION('center_axis',(0.,0.,-1.));
#15079=DIRECTION('ref_axis',(-1.,0.,0.));
#15080=DIRECTION('center_axis',(0.,0.,-1.));
#15081=DIRECTION('ref_axis',(-1.,0.,0.));
#15082=DIRECTION('center_axis',(0.,0.,-1.));
#15083=DIRECTION('ref_axis',(-1.,0.,0.));
#15084=DIRECTION('',(0.,0.,1.));
#15085=DIRECTION('center_axis',(0.,0.,-1.));
#15086=DIRECTION('ref_axis',(-1.,0.,0.));
#15087=DIRECTION('center_axis',(0.,0.,1.));
#15088=DIRECTION('ref_axis',(1.,0.,0.));
#15089=DIRECTION('center_axis',(0.,0.,1.));
#15090=DIRECTION('ref_axis',(1.,0.,0.));
#15091=DIRECTION('',(0.,0.,1.));
#15092=DIRECTION('center_axis',(0.,0.,1.));
#15093=DIRECTION('ref_axis',(1.,0.,0.));
#15094=DIRECTION('center_axis',(0.,0.,1.));
#15095=DIRECTION('ref_axis',(1.,0.,0.));
#15096=DIRECTION('center_axis',(0.,0.,1.));
#15097=DIRECTION('ref_axis',(1.,0.,0.));
#15098=DIRECTION('center_axis',(-1.22464679914735E-16,1.,0.));
#15099=DIRECTION('ref_axis',(-1.,-1.22464679914735E-16,0.));
#15100=DIRECTION('center_axis',(0.,0.,1.));
#15101=DIRECTION('ref_axis',(1.,0.,0.));
#15102=DIRECTION('center_axis',(0.,0.,1.));
#15103=DIRECTION('ref_axis',(1.,0.,0.));
#15104=DIRECTION('',(0.,0.,1.));
#15105=DIRECTION('center_axis',(0.,0.,1.));
#15106=DIRECTION('ref_axis',(1.,0.,0.));
#15107=DIRECTION('center_axis',(0.,0.,1.));
#15108=DIRECTION('ref_axis',(1.,0.,0.));
#15109=DIRECTION('center_axis',(0.,0.,1.));
#15110=DIRECTION('ref_axis',(1.,0.,0.));
#15111=DIRECTION('',(0.,0.,-1.));
#15112=DIRECTION('center_axis',(0.,0.,1.));
#15113=DIRECTION('ref_axis',(1.,0.,0.));
#15114=DIRECTION('center_axis',(0.,0.,-1.));
#15115=DIRECTION('ref_axis',(-1.,0.,0.));
#15116=DIRECTION('',(-0.707106781186546,8.65956056235491E-17,0.707106781186549));
#15117=DIRECTION('center_axis',(0.,0.,1.));
#15118=DIRECTION('ref_axis',(1.,0.,0.));
#15119=DIRECTION('center_axis',(0.,0.,1.));
#15120=DIRECTION('ref_axis',(1.,0.,0.));
#15121=DIRECTION('center_axis',(0.,0.,-1.));
#15122=DIRECTION('ref_axis',(-1.,0.,0.));
#15123=DIRECTION('center_axis',(0.,0.,1.));
#15124=DIRECTION('ref_axis',(1.,0.,0.));
#19778=CARTESIAN_POINT('',(0.,0.,0.));
#19779=CARTESIAN_POINT('Origin',(0.,0.,-3.46944695195361E-15));
#19780=CARTESIAN_POINT('',(-5.51648351648352,6.75574388101068E-16,1.11111111111111));
#19781=CARTESIAN_POINT('Origin',(0.,0.,1.11111111111111));
#19782=CARTESIAN_POINT('',(-5.51648351648352,-6.75574388101067E-16,-1.11111111111111));
#19783=CARTESIAN_POINT('Origin',(-6.,-7.34788079488412E-16,-3.46944695195361E-15));
#19784=CARTESIAN_POINT('Origin',(0.,0.,-1.11111111111111));
#19785=CARTESIAN_POINT('Origin',(0.,0.,2.5));
#19786=CARTESIAN_POINT('',(-4.,-4.89858719658941E-16,2.25));
#19787=CARTESIAN_POINT('Origin',(0.,0.,2.25));
#19788=CARTESIAN_POINT('',(-4.25,-5.20474889637625E-16,2.5));
#19789=CARTESIAN_POINT('',(-4.25,-5.20474889637625E-16,2.5));
#19790=CARTESIAN_POINT('Origin',(0.,0.,2.5));
#19791=CARTESIAN_POINT('Origin',(0.,0.,2.5));
#19792=CARTESIAN_POINT('',(4.,5.05166804648283E-16,-2.25));
#19793=CARTESIAN_POINT('',(-4.,-4.89858719658941E-16,-2.25));
#19794=CARTESIAN_POINT('Origin',(0.,0.,-2.25));
#19795=CARTESIAN_POINT('Origin',(0.,0.,-2.25));
#19796=CARTESIAN_POINT('',(-4.,-4.89858719658941E-16,2.5));
#19797=CARTESIAN_POINT('Origin',(0.,0.,-2.25));
#19798=CARTESIAN_POINT('',(4.25,-5.20474889637625E-16,-2.5));
#19799=CARTESIAN_POINT('',(4.,-4.89858719658941E-16,-2.25));
#19800=CARTESIAN_POINT('Origin',(0.,0.,-2.5));
#19801=CARTESIAN_POINT('Origin',(0.,0.,2.5));
#19802=CARTESIAN_POINT('',(-5.51648351648352,-6.75574388101067E-16,-2.5));
#19803=CARTESIAN_POINT('',(-5.51648351648352,-6.75574388101067E-16,2.5));
#19804=CARTESIAN_POINT('Origin',(0.,0.,-2.5));
#19805=CARTESIAN_POINT('Origin',(0.,0.,2.5));
#19806=CARTESIAN_POINT('',(-5.51648351648352,-6.75574388101067E-16,2.5));
#19807=CARTESIAN_POINT('Origin',(0.,0.,2.5));
#19808=CARTESIAN_POINT('',(-5.51648351648352,-6.75574388101067E-16,2.5));
#19809=CARTESIAN_POINT('Origin',(0.,5.51648351648352,2.5));
#19810=CARTESIAN_POINT('Origin',(0.,4.25,-2.5));
#19811=CARTESIAN_POINT('Origin',(0.,6.,0.));
#19812=CARTESIAN_POINT('',(-1.21175743903915,6.,9.08672536706121E-33));
#19813=CARTESIAN_POINT('',(1.21175743903915,6.,9.08672536706121E-33));
#19814=CARTESIAN_POINT('Origin',(0.,6.,0.));
#19815=CARTESIAN_POINT('Origin',(3.00000000000001,5.19615242270663,0.));
#19816=CARTESIAN_POINT('',(1.95058727456733,5.8020311422262,1.67904451446101E-32));
#19817=CARTESIAN_POINT('',(4.04941272543268,4.59027370318705,1.38300558951226E-33));
#19818=CARTESIAN_POINT('Origin',(3.00000000000001,5.19615242270663,0.));
#19819=CARTESIAN_POINT('Origin',(5.19615242270664,2.99999999999999,0.));
#19820=CARTESIAN_POINT('',(4.59027370318707,4.04941272543267,2.44941649221591E-32));
#19821=CARTESIAN_POINT('',(5.80203114222621,1.95058727456731,-6.32071418803668E-33));
#19822=CARTESIAN_POINT('Origin',(5.19615242270664,2.99999999999999,0.));
#19823=CARTESIAN_POINT('Origin',(6.,-2.08166817117217E-14,0.));
#19824=CARTESIAN_POINT('',(6.00000000000001,1.21175743903913,9.0867253670611E-33));
#19825=CARTESIAN_POINT('',(6.,-1.21175743903917,9.08672536706132E-33));
#19826=CARTESIAN_POINT('Origin',(6.,-2.08166817117217E-14,0.));
#19827=CARTESIAN_POINT('Origin',(5.19615242270662,-3.00000000000002,0.));
#19828=CARTESIAN_POINT('',(5.8020311422262,-1.95058727456735,-6.32071418803668E-33));
#19829=CARTESIAN_POINT('',(4.59027370318704,-4.0494127254327,2.44941649221591E-32));
#19830=CARTESIAN_POINT('Origin',(5.19615242270662,-3.00000000000002,0.));
#19831=CARTESIAN_POINT('Origin',(2.99999999999997,-5.19615242270665,0.));
#19832=CARTESIAN_POINT('',(4.04941272543265,-4.59027370318708,1.67904451446102E-32));
#19833=CARTESIAN_POINT('',(1.95058727456729,-5.80203114222622,1.38300558951227E-33));
#19834=CARTESIAN_POINT('Origin',(2.99999999999997,-5.19615242270665,0.));
#19835=CARTESIAN_POINT('Origin',(-4.16333634234434E-14,-6.,0.));
#19836=CARTESIAN_POINT('',(1.21175743903911,-6.00000000000001,9.08672536706099E-33));
#19837=CARTESIAN_POINT('',(-1.21175743903919,-5.99999999999999,9.08672536706142E-33));
#19838=CARTESIAN_POINT('Origin',(-4.16333634234434E-14,-6.,0.));
#19839=CARTESIAN_POINT('Origin',(-3.00000000000004,-5.19615242270661,0.));
#19840=CARTESIAN_POINT('',(-1.95058727456737,-5.80203114222619,3.2197884699708E-32));
#19841=CARTESIAN_POINT('',(-4.04941272543271,-4.59027370318703,-1.40244339655856E-32));
#19842=CARTESIAN_POINT('Origin',(-3.00000000000004,-5.19615242270661,0.));
#19843=CARTESIAN_POINT('Origin',(-5.19615242270666,-2.99999999999995,0.));
#19844=CARTESIAN_POINT('',(-4.5902737031871,-4.04941272543263,-6.32071418803668E-33));
#19845=CARTESIAN_POINT('',(-5.80203114222622,-1.95058727456727,2.44941649221591E-32));
#19846=CARTESIAN_POINT('Origin',(-5.19615242270666,-2.99999999999995,0.));
#19847=CARTESIAN_POINT('Origin',(-6.,6.24500451351651E-14,0.));
#19848=CARTESIAN_POINT('',(-6.00000000000001,-1.21175743903909,9.08672536706077E-33));
#19849=CARTESIAN_POINT('',(-5.99999999999999,1.21175743903921,9.08672536706164E-33));
#19850=CARTESIAN_POINT('Origin',(-6.,6.24500451351651E-14,0.));
#19851=CARTESIAN_POINT('Origin',(-5.1961524227066,3.00000000000006,0.));
#19852=CARTESIAN_POINT('',(-5.80203114222618,1.95058727456739,2.44941649221591E-32));
#19853=CARTESIAN_POINT('',(-4.59027370318701,4.04941272543273,-6.32071418803668E-33));
#19854=CARTESIAN_POINT('Origin',(-5.1961524227066,3.00000000000006,0.));
#19855=CARTESIAN_POINT('Origin',(-2.99999999999993,5.19615242270667,0.));
#19856=CARTESIAN_POINT('',(-4.04941272543262,4.59027370318711,1.38300558951226E-33));
#19857=CARTESIAN_POINT('',(-1.95058727456725,5.80203114222623,1.67904451446101E-32));
#19858=CARTESIAN_POINT('Origin',(-2.99999999999993,5.19615242270667,0.));
#19859=CARTESIAN_POINT('Origin',(0.,0.,2.5));
#19860=CARTESIAN_POINT('',(-6.48351648351648,-7.94001770875757E-16,2.375));
#19861=CARTESIAN_POINT('Origin',(0.,0.,2.375));
#19862=CARTESIAN_POINT('',(-6.48351648351648,-7.94001770875757E-16,1.21175743903915));
#19863=CARTESIAN_POINT('',(-6.48351648351648,-7.94001770875757E-16,2.5));
#19864=CARTESIAN_POINT('Origin',(0.,0.,1.21175743903915));
#19865=CARTESIAN_POINT('Origin',(0.,0.,2.5));
#19866=CARTESIAN_POINT('',(-5.51648351648352,-6.75574388101067E-16,1.21175743903915));
#19867=CARTESIAN_POINT('Origin',(0.,0.,1.21175743903915));
#19868=CARTESIAN_POINT('',(-5.51648351648352,-6.75574388101067E-16,2.375));
#19869=CARTESIAN_POINT('',(-5.51648351648352,-6.75574388101067E-16,2.5));
#19870=CARTESIAN_POINT('Origin',(0.,0.,2.375));
#19871=CARTESIAN_POINT('Origin',(0.,6.48351648351649,2.375));
#19872=CARTESIAN_POINT('Origin',(0.,6.48351648351649,1.21175743903915));
#19873=CARTESIAN_POINT('Origin',(0.,0.,2.5));
#19874=CARTESIAN_POINT('',(-6.48351648351649,-7.94001770875757E-16,-1.21175743903915));
#19875=CARTESIAN_POINT('Origin',(0.,0.,-1.21175743903915));
#19876=CARTESIAN_POINT('',(-6.48351648351649,-7.94001770875757E-16,-2.375));
#19877=CARTESIAN_POINT('',(-6.48351648351649,-7.94001770875757E-16,2.5));
#19878=CARTESIAN_POINT('Origin',(0.,0.,-2.375));
#19879=CARTESIAN_POINT('Origin',(0.,0.,2.5));
#19880=CARTESIAN_POINT('',(-5.51648351648352,-6.75574388101067E-16,-2.375));
#19881=CARTESIAN_POINT('Origin',(0.,0.,-2.375));
#19882=CARTESIAN_POINT('',(-5.51648351648352,-6.75574388101067E-16,-1.21175743903915));
#19883=CARTESIAN_POINT('',(-5.51648351648352,-6.75574388101067E-16,2.5));
#19884=CARTESIAN_POINT('Origin',(0.,0.,-1.21175743903915));
#19885=CARTESIAN_POINT('Origin',(0.,6.48351648351649,-2.375));
#19886=CARTESIAN_POINT('Origin',(0.,6.48351648351649,-1.21175743903915));
#19887=CARTESIAN_POINT('Origin',(0.,0.,-2.5));
#19888=CARTESIAN_POINT('',(9.,-1.10218211923262E-15,-2.5));
#19889=CARTESIAN_POINT('Origin',(0.,0.,-2.5));
#19890=CARTESIAN_POINT('',(9.,-1.10218211923262E-15,-1.4));
#19891=CARTESIAN_POINT('',(9.,-1.10218211923262E-15,-2.5));
#19892=CARTESIAN_POINT('Origin',(0.,0.,-1.4));
#19893=CARTESIAN_POINT('Origin',(0.,0.,2.5));
#19894=CARTESIAN_POINT('',(-6.48351648351648,-7.94001770875757E-16,1.11111111111111));
#19895=CARTESIAN_POINT('Origin',(0.,0.,1.11111111111111));
#19896=CARTESIAN_POINT('',(-6.48351648351648,-7.94001770875757E-16,2.5));
#19897=CARTESIAN_POINT('',(-6.48351648351648,-7.94001770875757E-16,2.5));
#19898=CARTESIAN_POINT('Origin',(0.,0.,2.5));
#19899=CARTESIAN_POINT('Origin',(0.,0.,0.));
#19900=CARTESIAN_POINT('',(-6.48351648351648,-7.94001770875757E-16,-1.11111111111111));
#19901=CARTESIAN_POINT('Origin',(0.,0.,-1.11111111111111));
#19902=CARTESIAN_POINT('Origin',(-6.,-7.34788079488412E-16,0.));
#19903=CARTESIAN_POINT('Origin',(0.,0.,2.5));
#19904=CARTESIAN_POINT('',(-6.48351648351648,-7.94001770875757E-16,-2.5));
#19905=CARTESIAN_POINT('Origin',(0.,0.,-2.5));
#19906=CARTESIAN_POINT('',(-6.48351648351648,-7.94001770875757E-16,2.5));
#19907=CARTESIAN_POINT('Origin',(0.,0.,2.5));
#19908=CARTESIAN_POINT('',(8.,9.79717439317883E-16,2.25));
#19909=CARTESIAN_POINT('',(-8.,-9.79717439317883E-16,2.25));
#19910=CARTESIAN_POINT('Origin',(0.,0.,2.25));
#19911=CARTESIAN_POINT('Origin',(0.,0.,2.25));
#19912=CARTESIAN_POINT('',(-8.,-9.79717439317883E-16,-1.4));
#19913=CARTESIAN_POINT('',(-8.,-9.79717439317883E-16,2.5));
#19914=CARTESIAN_POINT('Origin',(0.,0.,-1.4));
#19915=CARTESIAN_POINT('Origin',(0.,0.,2.25));
#19916=CARTESIAN_POINT('',(7.75,-9.49101269339199E-16,2.5));
#19917=CARTESIAN_POINT('',(8.,-9.79717439317883E-16,2.25));
#19918=CARTESIAN_POINT('Origin',(0.,0.,2.5));
#19919=CARTESIAN_POINT('Origin',(0.,7.75,-2.5));
#19920=CARTESIAN_POINT('Origin',(0.,7.75,2.5));
#19921=CARTESIAN_POINT('Origin',(0.,6.48351648351649,-1.4));
#20155=UNCERTAINTY_MEASURE_WITH_UNIT(LENGTH_MEASURE(0.01),#20177,
'DISTANCE_ACCURACY_VALUE',
'Maximum model space distance between geometric entities at asserted c
onnectivities');
#20160=UNCERTAINTY_MEASURE_WITH_UNIT(LENGTH_MEASURE(0.01),#20177,
'DISTANCE_ACCURACY_VALUE',
'Maximum model space distance between geometric entities at asserted c
onnectivities');
#20171=(
GEOMETRIC_REPRESENTATION_CONTEXT(3)
GLOBAL_UNCERTAINTY_ASSIGNED_CONTEXT((#20155))
GLOBAL_UNIT_ASSIGNED_CONTEXT((#20177,#20179,#20180))
REPRESENTATION_CONTEXT('','3D')
);
#20176=(
GEOMETRIC_REPRESENTATION_CONTEXT(3)
GLOBAL_UNCERTAINTY_ASSIGNED_CONTEXT((#20160))
GLOBAL_UNIT_ASSIGNED_CONTEXT((#20177,#20179,#20180))
REPRESENTATION_CONTEXT('','3D')
);
#20177=(
LENGTH_UNIT()
NAMED_UNIT(*)
SI_UNIT(.MILLI.,.METRE.)
);
#20179=(
NAMED_UNIT(*)
PLANE_ANGLE_UNIT()
SI_UNIT($,.RADIAN.)
);
#20180=(
NAMED_UNIT(*)
SI_UNIT($,.STERADIAN.)
SOLID_ANGLE_UNIT()
);
#20191=SHAPE_DEFINITION_REPRESENTATION(#20206,#20265);
#20206=PRODUCT_DEFINITION_SHAPE('',$,#20281);
#20265=SHAPE_REPRESENTATION('',(#12010),#20171);
#20270=PRODUCT_DEFINITION_CONTEXT('part definition',#20317,'design');
#20281=PRODUCT_DEFINITION('Flanged Bearing 8x16','Flanged Bearing 8x16',
#20296,#20270);
#20296=PRODUCT_DEFINITION_FORMATION('',$,#20329);
#20317=APPLICATION_CONTEXT(
'Core Data for Automotive Mechanical Design Process');
#20318=PRODUCT_CONTEXT('part definition',#20317,'mechanical');
#20329=PRODUCT('Flanged Bearing 8x16','Flanged Bearing 8x16',$,(#20318));
#20338=PRESENTATION_STYLE_ASSIGNMENT((#20343));
#20343=SURFACE_STYLE_USAGE(.BOTH.,#20348);
#20348=SURFACE_SIDE_STYLE('',(#20353));
#20353=SURFACE_STYLE_FILL_AREA(#20358);
#20358=FILL_AREA_STYLE('Opaque(122,133,145)',(#20363));
#20363=FILL_AREA_STYLE_COLOUR('Opaque(122,133,145)',#20368);
#20368=COLOUR_RGB('Opaque(122,133,145)',0.47843137254902,0.52156862745098,
0.568627450980392);
ENDSEC;
END-ISO-10303-21;
